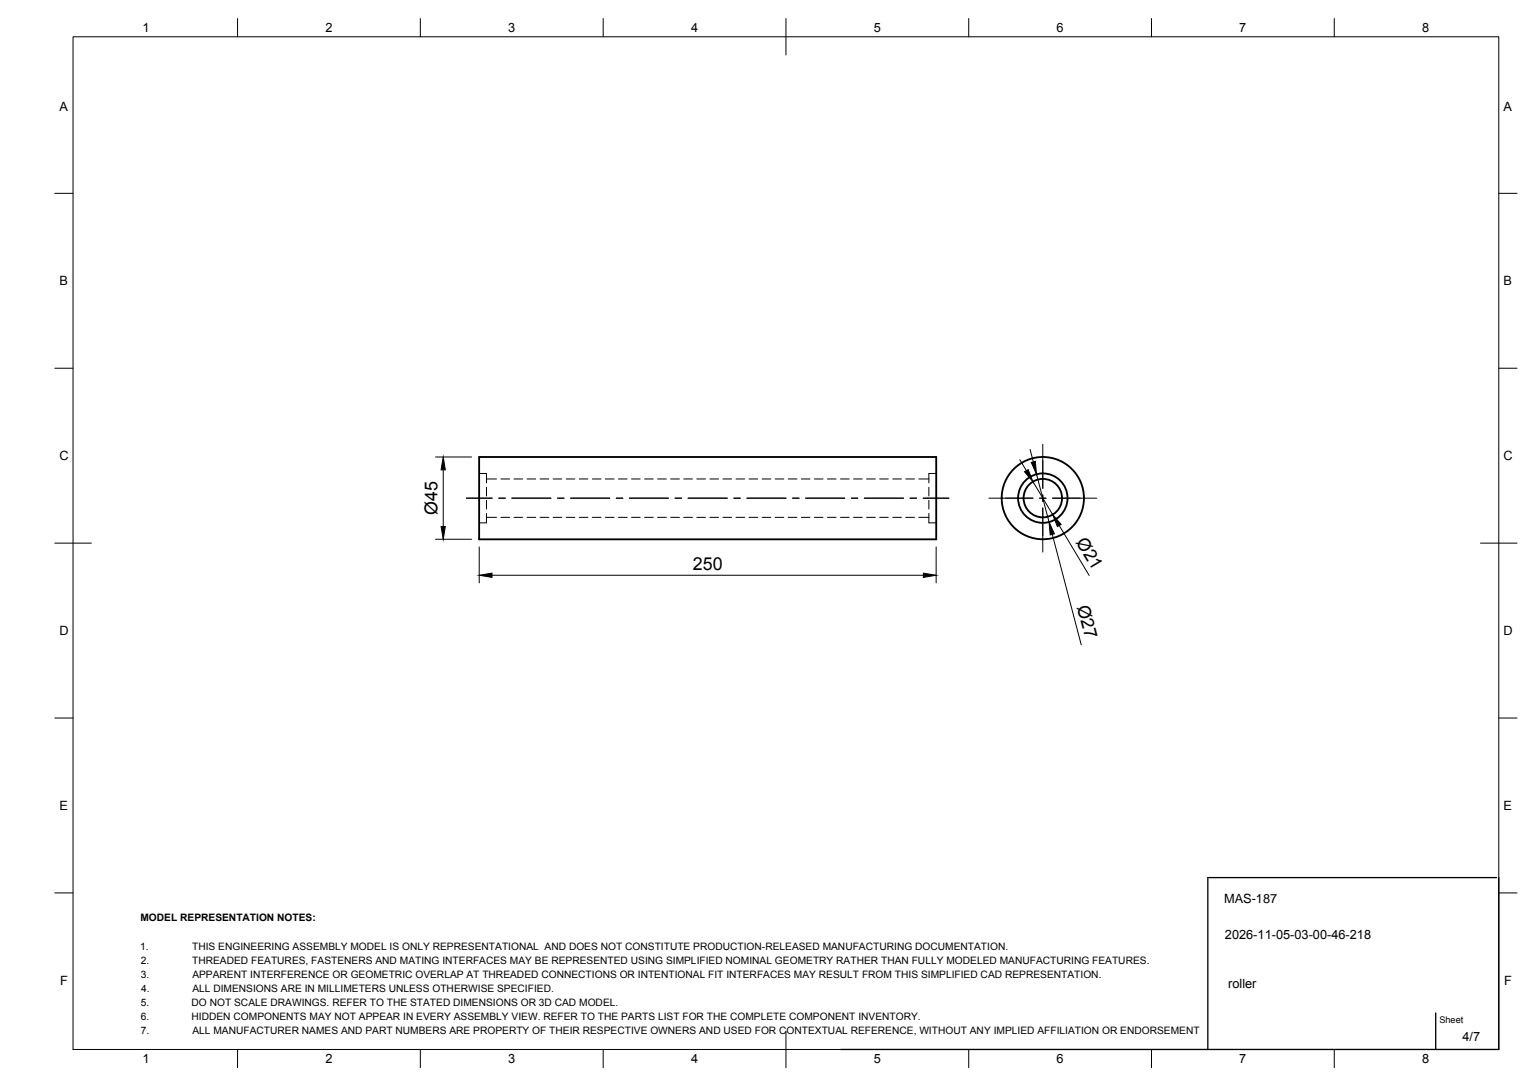
ISO-10303-21;
HEADER;
/* Generated by software containing ST-Developer
 * from STEP Tools, Inc. (www.steptools.com) 
 */

FILE_DESCRIPTION(
/* description */ ('STEP AP214'),
/* implementation_level */ '2;1');

FILE_NAME(
/* name */ 'roller.step',
/* time_stamp */ '2026-11-04T19:00:26-08:00',
/* author */ (''),
/* organization */ (''),
/* preprocessor_version */ 'ST-DEVELOPER v20.2',
/* originating_system */ 'Autodesk Translation Framework v15.17.0.0',
/* authorisation */ '');

FILE_SCHEMA (('AUTOMOTIVE_DESIGN { 1 0 10303 214 3 1 1 }'));
ENDSEC;

DATA;
#10=MECHANICAL_DESIGN_GEOMETRIC_PRESENTATION_REPRESENTATION('',(#275),#5689);
#261=SHAPE_REPRESENTATION_RELATIONSHIP('SRR','None',#5762,#268);
#268=ADVANCED_BREP_SHAPE_REPRESENTATION('',(#282),#5686);
#275=STYLED_ITEM('',(#5804),#282);
#282=MANIFOLD_SOLID_BREP('Body1',#2965);
#335=FACE_BOUND('',#760,.T.);
#336=FACE_BOUND('',#762,.T.);
#337=FACE_BOUND('',#764,.T.);
#338=FACE_BOUND('',#766,.T.);
#415=PLANE('',#3242);
#416=PLANE('',#3243);
#417=PLANE('',#3244);
#418=PLANE('',#3245);
#546=FACE_OUTER_BOUND('',#755,.T.);
#547=FACE_OUTER_BOUND('',#756,.T.);
#548=FACE_OUTER_BOUND('',#757,.T.);
#549=FACE_OUTER_BOUND('',#758,.T.);
#550=FACE_OUTER_BOUND('',#759,.T.);
#551=FACE_OUTER_BOUND('',#761,.T.);
#552=FACE_OUTER_BOUND('',#763,.T.);
#553=FACE_OUTER_BOUND('',#765,.T.);
#755=EDGE_LOOP('',(#2536,#2537,#2538,#2539));
#756=EDGE_LOOP('',(#2540,#2541,#2542,#2543));
#757=EDGE_LOOP('',(#2544,#2545,#2546,#2547));
#758=EDGE_LOOP('',(#2548,#2549,#2550,#2551));
#759=EDGE_LOOP('',(#2552));
#760=EDGE_LOOP('',(#2553));
#761=EDGE_LOOP('',(#2554));
#762=EDGE_LOOP('',(#2555));
#763=EDGE_LOOP('',(#2556));
#764=EDGE_LOOP('',(#2557));
#765=EDGE_LOOP('',(#2558));
#766=EDGE_LOOP('',(#2559));
#1006=LINE('',#4790,#1237);
#1007=LINE('',#4796,#1238);
#1008=LINE('',#4802,#1239);
#1009=LINE('',#4808,#1240);
#1237=VECTOR('',#3929,13.5);
#1238=VECTOR('',#3936,13.5);
#1239=VECTOR('',#3943,22.5);
#1240=VECTOR('',#3950,10.5);
#1354=CIRCLE('',#3231,13.5);
#1355=CIRCLE('',#3232,13.5);
#1356=CIRCLE('',#3234,13.5);
#1357=CIRCLE('',#3235,13.5);
#1358=CIRCLE('',#3237,22.5);
#1359=CIRCLE('',#3238,22.5);
#1360=CIRCLE('',#3240,10.5);
#1361=CIRCLE('',#3241,10.5);
#1563=VERTEX_POINT('',#4787);
#1564=VERTEX_POINT('',#4789);
#1565=VERTEX_POINT('',#4793);
#1566=VERTEX_POINT('',#4795);
#1567=VERTEX_POINT('',#4799);
#1568=VERTEX_POINT('',#4801);
#1569=VERTEX_POINT('',#4805);
#1570=VERTEX_POINT('',#4807);
#1896=EDGE_CURVE('',#1563,#1563,#1354,.T.);
#1897=EDGE_CURVE('',#1563,#1564,#1006,.T.);
#1898=EDGE_CURVE('',#1564,#1564,#1355,.T.);
#1899=EDGE_CURVE('',#1565,#1565,#1356,.T.);
#1900=EDGE_CURVE('',#1565,#1566,#1007,.T.);
#1901=EDGE_CURVE('',#1566,#1566,#1357,.T.);
#1902=EDGE_CURVE('',#1567,#1567,#1358,.T.);
#1903=EDGE_CURVE('',#1567,#1568,#1008,.T.);
#1904=EDGE_CURVE('',#1568,#1568,#1359,.T.);
#1905=EDGE_CURVE('',#1569,#1569,#1360,.T.);
#1906=EDGE_CURVE('',#1569,#1570,#1009,.T.);
#1907=EDGE_CURVE('',#1570,#1570,#1361,.T.);
#2536=ORIENTED_EDGE('',*,*,#1896,.T.);
#2537=ORIENTED_EDGE('',*,*,#1897,.T.);
#2538=ORIENTED_EDGE('',*,*,#1898,.F.);
#2539=ORIENTED_EDGE('',*,*,#1897,.F.);
#2540=ORIENTED_EDGE('',*,*,#1899,.F.);
#2541=ORIENTED_EDGE('',*,*,#1900,.T.);
#2542=ORIENTED_EDGE('',*,*,#1901,.T.);
#2543=ORIENTED_EDGE('',*,*,#1900,.F.);
#2544=ORIENTED_EDGE('',*,*,#1902,.T.);
#2545=ORIENTED_EDGE('',*,*,#1903,.T.);
#2546=ORIENTED_EDGE('',*,*,#1904,.F.);
#2547=ORIENTED_EDGE('',*,*,#1903,.F.);
#2548=ORIENTED_EDGE('',*,*,#1905,.T.);
#2549=ORIENTED_EDGE('',*,*,#1906,.T.);
#2550=ORIENTED_EDGE('',*,*,#1907,.T.);
#2551=ORIENTED_EDGE('',*,*,#1906,.F.);
#2552=ORIENTED_EDGE('',*,*,#1904,.T.);
#2553=ORIENTED_EDGE('',*,*,#1901,.F.);
#2554=ORIENTED_EDGE('',*,*,#1902,.F.);
#2555=ORIENTED_EDGE('',*,*,#1898,.T.);
#2556=ORIENTED_EDGE('',*,*,#1899,.T.);
#2557=ORIENTED_EDGE('',*,*,#1905,.F.);
#2558=ORIENTED_EDGE('',*,*,#1896,.F.);
#2559=ORIENTED_EDGE('',*,*,#1907,.F.);
#2794=CYLINDRICAL_SURFACE('',#3230,13.5);
#2795=CYLINDRICAL_SURFACE('',#3233,13.5);
#2796=CYLINDRICAL_SURFACE('',#3236,22.5);
#2797=CYLINDRICAL_SURFACE('',#3239,10.5);
#2906=ADVANCED_FACE('',(#546),#2794,.F.);
#2907=ADVANCED_FACE('',(#547),#2795,.F.);
#2908=ADVANCED_FACE('',(#548),#2796,.T.);
#2909=ADVANCED_FACE('',(#549),#2797,.F.);
#2910=ADVANCED_FACE('',(#550,#335),#415,.T.);
#2911=ADVANCED_FACE('',(#551,#336),#416,.F.);
#2912=ADVANCED_FACE('',(#552,#337),#417,.T.);
#2913=ADVANCED_FACE('',(#553,#338),#418,.T.);
#2965=CLOSED_SHELL('',(#2906,#2907,#2908,#2909,#2910,#2911,#2912,#2913));
#3229=AXIS2_PLACEMENT_3D('',#4785,#3923,#3924);
#3230=AXIS2_PLACEMENT_3D('',#4786,#3925,#3926);
#3231=AXIS2_PLACEMENT_3D('',#4788,#3927,#3928);
#3232=AXIS2_PLACEMENT_3D('',#4791,#3930,#3931);
#3233=AXIS2_PLACEMENT_3D('',#4792,#3932,#3933);
#3234=AXIS2_PLACEMENT_3D('',#4794,#3934,#3935);
#3235=AXIS2_PLACEMENT_3D('',#4797,#3937,#3938);
#3236=AXIS2_PLACEMENT_3D('',#4798,#3939,#3940);
#3237=AXIS2_PLACEMENT_3D('',#4800,#3941,#3942);
#3238=AXIS2_PLACEMENT_3D('',#4803,#3944,#3945);
#3239=AXIS2_PLACEMENT_3D('',#4804,#3946,#3947);
#3240=AXIS2_PLACEMENT_3D('',#4806,#3948,#3949);
#3241=AXIS2_PLACEMENT_3D('',#4809,#3951,#3952);
#3242=AXIS2_PLACEMENT_3D('',#4810,#3953,#3954);
#3243=AXIS2_PLACEMENT_3D('',#4811,#3955,#3956);
#3244=AXIS2_PLACEMENT_3D('',#4812,#3957,#3958);
#3245=AXIS2_PLACEMENT_3D('',#4813,#3959,#3960);
#3923=DIRECTION('axis',(0.,0.,1.));
#3924=DIRECTION('refdir',(1.,0.,0.));
#3925=DIRECTION('center_axis',(0.,0.,-1.));
#3926=DIRECTION('ref_axis',(-1.,0.,0.));
#3927=DIRECTION('center_axis',(0.,0.,1.));
#3928=DIRECTION('ref_axis',(1.,0.,0.));
#3929=DIRECTION('',(0.,0.,-1.));
#3930=DIRECTION('center_axis',(0.,0.,1.));
#3931=DIRECTION('ref_axis',(1.,0.,0.));
#3932=DIRECTION('center_axis',(0.,0.,1.));
#3933=DIRECTION('ref_axis',(1.,0.,0.));
#3934=DIRECTION('center_axis',(0.,0.,1.));
#3935=DIRECTION('ref_axis',(1.,0.,0.));
#3936=DIRECTION('',(0.,0.,1.));
#3937=DIRECTION('center_axis',(0.,0.,1.));
#3938=DIRECTION('ref_axis',(1.,0.,0.));
#3939=DIRECTION('center_axis',(0.,0.,-1.));
#3940=DIRECTION('ref_axis',(-1.,0.,0.));
#3941=DIRECTION('center_axis',(0.,0.,1.));
#3942=DIRECTION('ref_axis',(1.,0.,0.));
#3943=DIRECTION('',(0.,0.,1.));
#3944=DIRECTION('center_axis',(0.,0.,1.));
#3945=DIRECTION('ref_axis',(1.,0.,0.));
#3946=DIRECTION('center_axis',(0.,0.,-1.));
#3947=DIRECTION('ref_axis',(-1.,0.,0.));
#3948=DIRECTION('center_axis',(0.,0.,1.));
#3949=DIRECTION('ref_axis',(1.,0.,0.));
#3950=DIRECTION('',(0.,0.,-1.));
#3951=DIRECTION('center_axis',(0.,0.,-1.));
#3952=DIRECTION('ref_axis',(-1.,0.,0.));
#3953=DIRECTION('center_axis',(0.,0.,1.));
#3954=DIRECTION('ref_axis',(1.,0.,0.));
#3955=DIRECTION('center_axis',(0.,0.,1.));
#3956=DIRECTION('ref_axis',(1.,0.,0.));
#3957=DIRECTION('center_axis',(0.,0.,1.));
#3958=DIRECTION('ref_axis',(1.,0.,0.));
#3959=DIRECTION('center_axis',(0.,0.,-1.));
#3960=DIRECTION('ref_axis',(1.,0.,0.));
#4785=CARTESIAN_POINT('',(0.,0.,0.));
#4786=CARTESIAN_POINT('Origin',(0.,0.,-121.));
#4787=CARTESIAN_POINT('',(13.5,-1.65327317884893E-15,-121.));
#4788=CARTESIAN_POINT('Origin',(0.,0.,-121.));
#4789=CARTESIAN_POINT('',(13.5,-1.65327317884893E-15,-125.));
#4790=CARTESIAN_POINT('',(13.5,-1.65327317884893E-15,-121.));
#4791=CARTESIAN_POINT('Origin',(0.,0.,-125.));
#4792=CARTESIAN_POINT('Origin',(0.,0.,121.));
#4793=CARTESIAN_POINT('',(-13.5,-1.65327317884893E-15,121.));
#4794=CARTESIAN_POINT('Origin',(0.,0.,121.));
#4795=CARTESIAN_POINT('',(-13.5,-1.65327317884893E-15,125.));
#4796=CARTESIAN_POINT('',(-13.5,-1.65327317884893E-15,121.));
#4797=CARTESIAN_POINT('Origin',(0.,0.,125.));
#4798=CARTESIAN_POINT('Origin',(0.,0.,125.));
#4799=CARTESIAN_POINT('',(22.5,-2.75545529808155E-15,-125.));
#4800=CARTESIAN_POINT('Origin',(0.,0.,-125.));
#4801=CARTESIAN_POINT('',(22.5,-2.75545529808155E-15,125.));
#4802=CARTESIAN_POINT('',(22.5,-2.75545529808155E-15,125.));
#4803=CARTESIAN_POINT('Origin',(0.,0.,125.));
#4804=CARTESIAN_POINT('Origin',(0.,0.,125.));
#4805=CARTESIAN_POINT('',(10.5,-1.28587913910472E-15,121.));
#4806=CARTESIAN_POINT('Origin',(0.,0.,121.));
#4807=CARTESIAN_POINT('',(10.5,-1.28587913910472E-15,-121.));
#4808=CARTESIAN_POINT('',(10.5,-1.28587913910472E-15,125.));
#4809=CARTESIAN_POINT('Origin',(0.,0.,-121.));
#4810=CARTESIAN_POINT('Origin',(0.,0.,125.));
#4811=CARTESIAN_POINT('Origin',(0.,0.,-125.));
#4812=CARTESIAN_POINT('Origin',(0.,0.,121.));
#4813=CARTESIAN_POINT('Origin',(0.,0.,-121.));
#5677=UNCERTAINTY_MEASURE_WITH_UNIT(LENGTH_MEASURE(0.01),#5690,
'DISTANCE_ACCURACY_VALUE',
'Maximum model space distance between geometric entities at asserted c
onnectivities');
#5680=UNCERTAINTY_MEASURE_WITH_UNIT(LENGTH_MEASURE(0.01),#5690,
'DISTANCE_ACCURACY_VALUE',
'Maximum model space distance between geometric entities at asserted c
onnectivities');
#5686=(
GEOMETRIC_REPRESENTATION_CONTEXT(3)
GLOBAL_UNCERTAINTY_ASSIGNED_CONTEXT((#5677))
GLOBAL_UNIT_ASSIGNED_CONTEXT((#5690,#5692,#5693))
REPRESENTATION_CONTEXT('','3D')
);
#5689=(
GEOMETRIC_REPRESENTATION_CONTEXT(3)
GLOBAL_UNCERTAINTY_ASSIGNED_CONTEXT((#5680))
GLOBAL_UNIT_ASSIGNED_CONTEXT((#5690,#5692,#5693))
REPRESENTATION_CONTEXT('','3D')
);
#5690=(
LENGTH_UNIT()
NAMED_UNIT(*)
SI_UNIT(.MILLI.,.METRE.)
);
#5692=(
NAMED_UNIT(*)
PLANE_ANGLE_UNIT()
SI_UNIT($,.RADIAN.)
);
#5693=(
NAMED_UNIT(*)
SI_UNIT($,.STERADIAN.)
SOLID_ANGLE_UNIT()
);
#5699=SHAPE_DEFINITION_REPRESENTATION(#5707,#5762);
#5707=PRODUCT_DEFINITION_SHAPE('',$,#5771);
#5762=SHAPE_REPRESENTATION('',(#3229),#5686);
#5765=PRODUCT_DEFINITION_CONTEXT('part definition',#5791,'design');
#5771=PRODUCT_DEFINITION('roller','roller',#5779,#5765);
#5779=PRODUCT_DEFINITION_FORMATION('',$,#5798);
#5791=APPLICATION_CONTEXT(
'Core Data for Automotive Mechanical Design Process');
#5792=PRODUCT_CONTEXT('part definition',#5791,'mechanical');
#5798=PRODUCT('roller','roller',$,(#5792));
#5804=PRESENTATION_STYLE_ASSIGNMENT((#5810));
#5810=SURFACE_STYLE_USAGE(.BOTH.,#5816);
#5816=SURFACE_SIDE_STYLE('',(#5822));
#5822=SURFACE_STYLE_FILL_AREA(#5828);
#5828=FILL_AREA_STYLE('Opaque(61,176,222)',(#5834));
#5834=FILL_AREA_STYLE_COLOUR('Opaque(61,176,222)',#5840);
#5840=COLOUR_RGB('Opaque(61,176,222)',0.23921568627451,0.690196078431373,
0.870588235294118);
ENDSEC;
END-ISO-10303-21;
